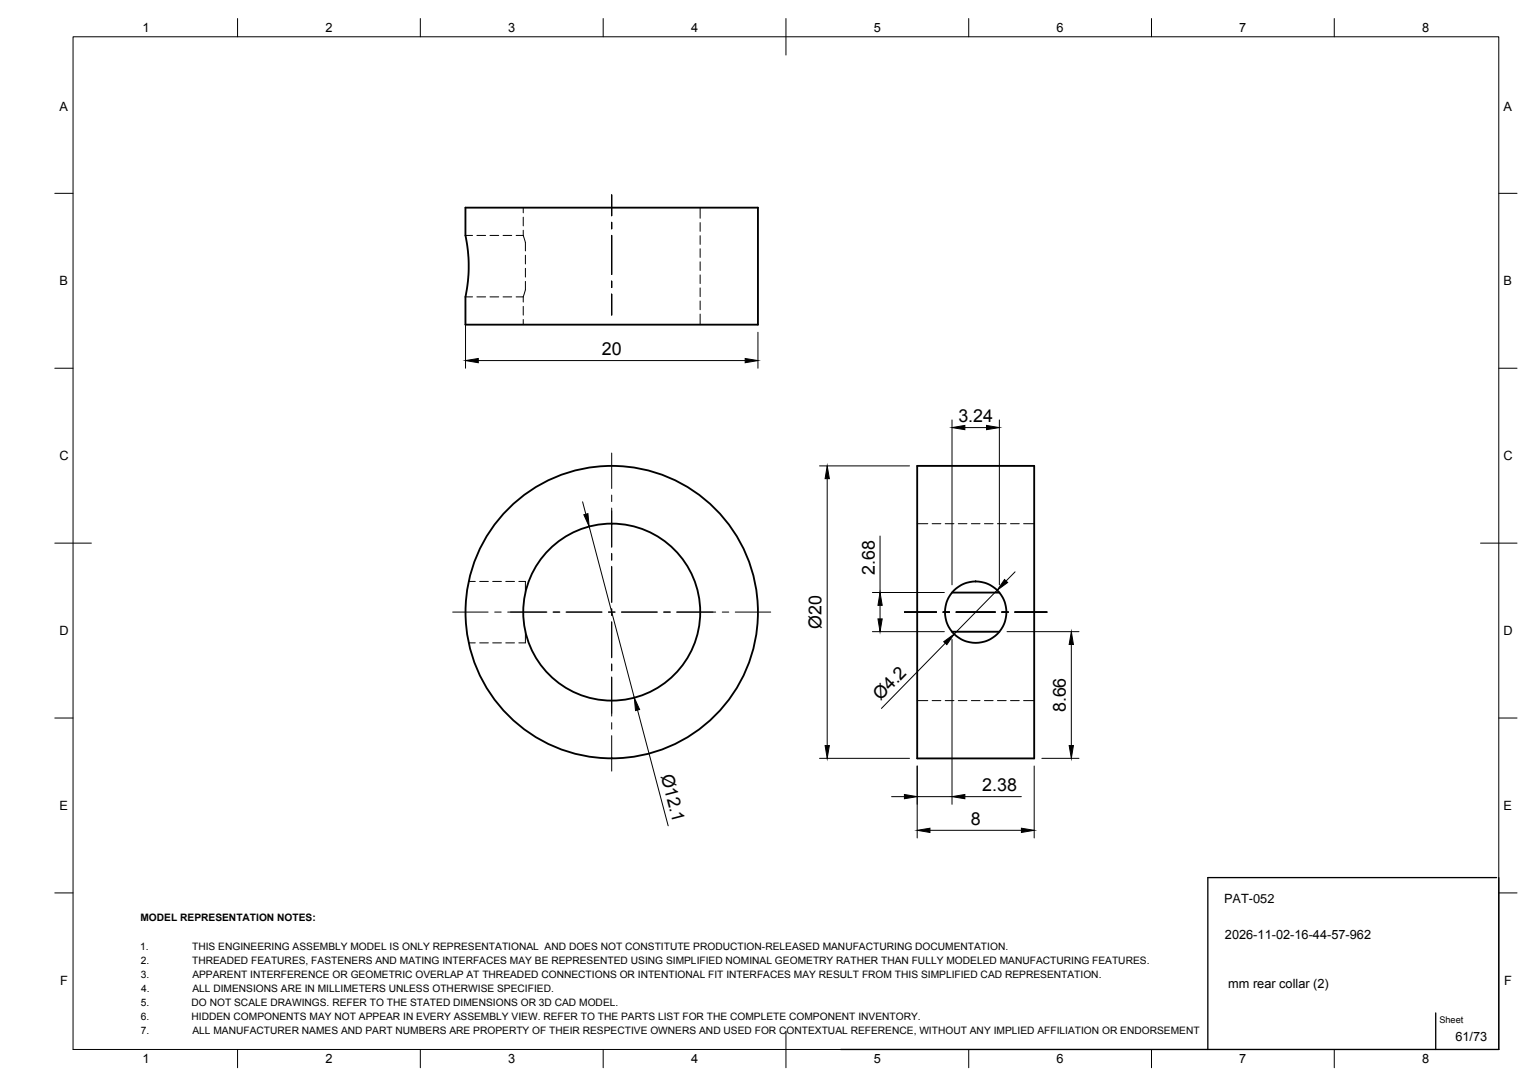
ISO-10303-21;
HEADER;
/* Generated by software containing ST-Developer
 * from STEP Tools, Inc. (www.steptools.com) 
 */

FILE_DESCRIPTION(
/* description */ ('Hand-crank gear train demonstrator'),
/* implementation_level */ '2;1');

FILE_NAME(
/* name */ 'mm rear collar (2).step',
/* time_stamp */ '2026-10-28T03:22:13-07:00',
/* author */ (''),
/* organization */ (''),
/* preprocessor_version */ 'ST-DEVELOPER v20.2',
/* originating_system */ 'Autodesk Translation Framework v15.17.0.0',
/* authorisation */ '');

FILE_SCHEMA (('AUTOMOTIVE_DESIGN { 1 0 10303 214 3 1 1 }'));
ENDSEC;

DATA;
#10=MECHANICAL_DESIGN_GEOMETRIC_PRESENTATION_REPRESENTATION('',(#1251),#62758);
#899=B_SPLINE_CURVE_WITH_KNOTS('',3,(#26683,#26684,#26685,#26686,#26687,
#26688,#26689,#26690,#26691,#26692),.UNSPECIFIED.,.F.,.F.,(4,2,2,2,4),(0.81808890434921,
0.878131747417167,0.957937926194039,1.03774410497091,1.09778694803887),
 .UNSPECIFIED.);
#900=B_SPLINE_CURVE_WITH_KNOTS('',3,(#26698,#26699,#26700,#26701,#26702,
#26703,#26704,#26705,#26706,#26707,#26708,#26709,#26710,#26711,#26712,#26713,
#26714,#26715),.UNSPECIFIED.,.F.,.F.,(4,2,2,2,2,2,2,2,4),(0.,0.0793616477694788,
0.158723295538958,0.238079516586307,0.317435737633657,0.396791958681007,
0.476148179728357,0.555509827497836,0.634871475267315),.UNSPECIFIED.);
#901=B_SPLINE_CURVE_WITH_KNOTS('',3,(#26716,#26717,#26718,#26719,#26720,
#26721,#26722,#26723,#26724,#26725,#26726,#26727,#26728,#26729,#26730,#26731,
#26732,#26733),.UNSPECIFIED.,.F.,.F.,(4,2,2,2,2,2,2,2,4),(0.634871475267315,
0.714233123036793,0.793594770806272,0.872950991853622,0.952307212900972,
1.03166343394832,1.11101965499567,1.19038130276515,1.26974295053463),
 .UNSPECIFIED.);
#902=B_SPLINE_CURVE_WITH_KNOTS('',3,(#26736,#26737,#26738,#26739,#26740,
#26741,#26742,#26743,#26744,#26745),.UNSPECIFIED.,.F.,.F.,(4,2,2,2,4),(0.17946362021985,
0.239506463287808,0.31931264206468,0.399118820841551,0.459161663909509),
 .UNSPECIFIED.);
#1108=SHAPE_REPRESENTATION_RELATIONSHIP('SRR','None',#63085,#1172);
#1172=ADVANCED_BREP_SHAPE_REPRESENTATION('',(#1326),#62739);
#1251=STYLED_ITEM('',(#63448),#1326);
#1326=MANIFOLD_SOLID_BREP('Body1',#16435);
#1594=FACE_BOUND('',#3879,.T.);
#1595=FACE_BOUND('',#3881,.T.);
#1596=FACE_BOUND('',#3883,.T.);
#1597=FACE_BOUND('',#3885,.T.);
#1971=PLANE('',#18248);
#1972=PLANE('',#18253);
#1973=PLANE('',#18260);
#1974=PLANE('',#18261);
#2687=FACE_OUTER_BOUND('',#3875,.T.);
#2688=FACE_OUTER_BOUND('',#3876,.T.);
#2689=FACE_OUTER_BOUND('',#3877,.T.);
#2690=FACE_OUTER_BOUND('',#3878,.T.);
#2691=FACE_OUTER_BOUND('',#3880,.T.);
#2692=FACE_OUTER_BOUND('',#3882,.T.);
#2693=FACE_OUTER_BOUND('',#3884,.T.);
#3875=EDGE_LOOP('',(#13211,#13212));
#3876=EDGE_LOOP('',(#13213,#13214,#13215,#13216,#13217,#13218,#13219,#13220,
#13221));
#3877=EDGE_LOOP('',(#13222,#13223,#13224));
#3878=EDGE_LOOP('',(#13225,#13226,#13227,#13228));
#3879=EDGE_LOOP('',(#13229,#13230,#13231,#13232));
#3880=EDGE_LOOP('',(#13233,#13234,#13235,#13236));
#3881=EDGE_LOOP('',(#13237,#13238));
#3882=EDGE_LOOP('',(#13239));
#3883=EDGE_LOOP('',(#13240));
#3884=EDGE_LOOP('',(#13241));
#3885=EDGE_LOOP('',(#13242));
#4973=LINE('',#26679,#6105);
#4974=LINE('',#26696,#6106);
#4975=LINE('',#26747,#6107);
#4976=LINE('',#26752,#6108);
#4977=LINE('',#26758,#6109);
#6105=VECTOR('',#21700,1.);
#6106=VECTOR('',#21707,0.210000000000001);
#6107=VECTOR('',#21712,1.);
#6108=VECTOR('',#21717,0.605);
#6109=VECTOR('',#21724,1.);
#7011=CIRCLE('',#18249,0.210000000000001);
#7012=CIRCLE('',#18251,0.210000000000001);
#7013=CIRCLE('',#18252,0.210000000000001);
#7014=CIRCLE('',#18255,0.605);
#7015=CIRCLE('',#18256,0.605);
#7016=CIRCLE('',#18258,1.);
#7017=CIRCLE('',#18259,1.);
#8018=VERTEX_POINT('',#26677);
#8019=VERTEX_POINT('',#26678);
#8020=VERTEX_POINT('',#26682);
#8021=VERTEX_POINT('',#26693);
#8022=VERTEX_POINT('',#26695);
#8023=VERTEX_POINT('',#26697);
#8024=VERTEX_POINT('',#26734);
#8025=VERTEX_POINT('',#26749);
#8026=VERTEX_POINT('',#26751);
#8027=VERTEX_POINT('',#26755);
#8028=VERTEX_POINT('',#26757);
#9857=EDGE_CURVE('',#8018,#8019,#4973,.T.);
#9858=EDGE_CURVE('',#8018,#8019,#7011,.T.);
#9859=EDGE_CURVE('',#8020,#8018,#899,.T.);
#9860=EDGE_CURVE('',#8021,#8020,#7012,.T.);
#9861=EDGE_CURVE('',#8021,#8022,#4974,.T.);
#9862=EDGE_CURVE('',#8023,#8022,#900,.T.);
#9863=EDGE_CURVE('',#8022,#8023,#901,.T.);
#9864=EDGE_CURVE('',#8024,#8021,#7013,.T.);
#9865=EDGE_CURVE('',#8019,#8024,#902,.T.);
#9866=EDGE_CURVE('',#8024,#8020,#4975,.T.);
#9867=EDGE_CURVE('',#8025,#8025,#7014,.T.);
#9868=EDGE_CURVE('',#8025,#8026,#4976,.T.);
#9869=EDGE_CURVE('',#8026,#8026,#7015,.T.);
#9870=EDGE_CURVE('',#8027,#8027,#7016,.T.);
#9871=EDGE_CURVE('',#8027,#8028,#4977,.T.);
#9872=EDGE_CURVE('',#8028,#8028,#7017,.T.);
#13211=ORIENTED_EDGE('',*,*,#9857,.F.);
#13212=ORIENTED_EDGE('',*,*,#9858,.T.);
#13213=ORIENTED_EDGE('',*,*,#9859,.F.);
#13214=ORIENTED_EDGE('',*,*,#9860,.F.);
#13215=ORIENTED_EDGE('',*,*,#9861,.T.);
#13216=ORIENTED_EDGE('',*,*,#9862,.F.);
#13217=ORIENTED_EDGE('',*,*,#9863,.F.);
#13218=ORIENTED_EDGE('',*,*,#9861,.F.);
#13219=ORIENTED_EDGE('',*,*,#9864,.F.);
#13220=ORIENTED_EDGE('',*,*,#9865,.F.);
#13221=ORIENTED_EDGE('',*,*,#9858,.F.);
#13222=ORIENTED_EDGE('',*,*,#9866,.F.);
#13223=ORIENTED_EDGE('',*,*,#9864,.T.);
#13224=ORIENTED_EDGE('',*,*,#9860,.T.);
#13225=ORIENTED_EDGE('',*,*,#9867,.F.);
#13226=ORIENTED_EDGE('',*,*,#9868,.T.);
#13227=ORIENTED_EDGE('',*,*,#9869,.T.);
#13228=ORIENTED_EDGE('',*,*,#9868,.F.);
#13229=ORIENTED_EDGE('',*,*,#9865,.T.);
#13230=ORIENTED_EDGE('',*,*,#9866,.T.);
#13231=ORIENTED_EDGE('',*,*,#9859,.T.);
#13232=ORIENTED_EDGE('',*,*,#9857,.T.);
#13233=ORIENTED_EDGE('',*,*,#9870,.F.);
#13234=ORIENTED_EDGE('',*,*,#9871,.T.);
#13235=ORIENTED_EDGE('',*,*,#9872,.T.);
#13236=ORIENTED_EDGE('',*,*,#9871,.F.);
#13237=ORIENTED_EDGE('',*,*,#9862,.T.);
#13238=ORIENTED_EDGE('',*,*,#9863,.T.);
#13239=ORIENTED_EDGE('',*,*,#9870,.T.);
#13240=ORIENTED_EDGE('',*,*,#9867,.T.);
#13241=ORIENTED_EDGE('',*,*,#9872,.F.);
#13242=ORIENTED_EDGE('',*,*,#9869,.F.);
#15339=CYLINDRICAL_SURFACE('',#18250,0.210000000000001);
#15340=CYLINDRICAL_SURFACE('',#18254,0.605);
#15341=CYLINDRICAL_SURFACE('',#18257,1.);
#15997=ADVANCED_FACE('',(#2687),#1971,.T.);
#15998=ADVANCED_FACE('',(#2688),#15339,.F.);
#15999=ADVANCED_FACE('',(#2689),#1972,.T.);
#16000=ADVANCED_FACE('',(#2690,#1594),#15340,.F.);
#16001=ADVANCED_FACE('',(#2691,#1595),#15341,.T.);
#16002=ADVANCED_FACE('',(#2692,#1596),#1973,.T.);
#16003=ADVANCED_FACE('',(#2693,#1597),#1974,.F.);
#16435=CLOSED_SHELL('',(#15997,#15998,#15999,#16000,#16001,#16002,#16003));
#18247=AXIS2_PLACEMENT_3D('',#26675,#21696,#21697);
#18248=AXIS2_PLACEMENT_3D('',#26676,#21698,#21699);
#18249=AXIS2_PLACEMENT_3D('',#26680,#21701,#21702);
#18250=AXIS2_PLACEMENT_3D('',#26681,#21703,#21704);
#18251=AXIS2_PLACEMENT_3D('',#26694,#21705,#21706);
#18252=AXIS2_PLACEMENT_3D('',#26735,#21708,#21709);
#18253=AXIS2_PLACEMENT_3D('',#26746,#21710,#21711);
#18254=AXIS2_PLACEMENT_3D('',#26748,#21713,#21714);
#18255=AXIS2_PLACEMENT_3D('',#26750,#21715,#21716);
#18256=AXIS2_PLACEMENT_3D('',#26753,#21718,#21719);
#18257=AXIS2_PLACEMENT_3D('',#26754,#21720,#21721);
#18258=AXIS2_PLACEMENT_3D('',#26756,#21722,#21723);
#18259=AXIS2_PLACEMENT_3D('',#26759,#21725,#21726);
#18260=AXIS2_PLACEMENT_3D('',#26760,#21727,#21728);
#18261=AXIS2_PLACEMENT_3D('',#26761,#21729,#21730);
#21696=DIRECTION('axis',(0.,0.,1.));
#21697=DIRECTION('refdir',(1.,0.,0.));
#21698=DIRECTION('center_axis',(0.,0.,1.));
#21699=DIRECTION('ref_axis',(1.,0.,0.));
#21700=DIRECTION('',(0.,1.,0.));
#21701=DIRECTION('center_axis',(0.,0.,1.));
#21702=DIRECTION('ref_axis',(1.,0.,0.));
#21703=DIRECTION('center_axis',(0.,0.,1.));
#21704=DIRECTION('ref_axis',(1.,0.,0.));
#21705=DIRECTION('center_axis',(0.,0.,1.));
#21706=DIRECTION('ref_axis',(1.,0.,0.));
#21707=DIRECTION('',(0.,0.,1.));
#21708=DIRECTION('center_axis',(0.,0.,1.));
#21709=DIRECTION('ref_axis',(1.,0.,0.));
#21710=DIRECTION('center_axis',(0.,0.,1.));
#21711=DIRECTION('ref_axis',(1.,0.,0.));
#21712=DIRECTION('',(0.,-1.,0.));
#21713=DIRECTION('center_axis',(0.,1.,0.));
#21714=DIRECTION('ref_axis',(1.,0.,0.));
#21715=DIRECTION('center_axis',(0.,-1.,0.));
#21716=DIRECTION('ref_axis',(1.,0.,0.));
#21717=DIRECTION('',(0.,-1.,0.));
#21718=DIRECTION('center_axis',(0.,-1.,0.));
#21719=DIRECTION('ref_axis',(1.,0.,0.));
#21720=DIRECTION('center_axis',(0.,1.,0.));
#21721=DIRECTION('ref_axis',(1.,0.,0.));
#21722=DIRECTION('center_axis',(0.,1.,0.));
#21723=DIRECTION('ref_axis',(1.,0.,0.));
#21724=DIRECTION('',(0.,-1.,0.));
#21725=DIRECTION('center_axis',(0.,1.,0.));
#21726=DIRECTION('ref_axis',(1.,0.,0.));
#21727=DIRECTION('center_axis',(0.,1.,0.));
#21728=DIRECTION('ref_axis',(1.,0.,0.));
#21729=DIRECTION('center_axis',(0.,1.,0.));
#21730=DIRECTION('ref_axis',(1.,0.,0.));
#26675=CARTESIAN_POINT('',(0.,0.,0.));
#26676=CARTESIAN_POINT('Origin',(12.,-3.2,9.59));
#26677=CARTESIAN_POINT('',(12.1338842783899,-3.36178689687366,9.59));
#26678=CARTESIAN_POINT('',(12.1338842783899,-3.03821310312634,9.59));
#26679=CARTESIAN_POINT('',(12.13388427839,-3.6,9.59));
#26680=CARTESIAN_POINT('Origin',(12.,-3.2,9.59));
#26681=CARTESIAN_POINT('Origin',(12.,-3.2,9.59));
#26682=CARTESIAN_POINT('',(11.8661157216101,-3.36178689687366,9.59));
#26683=CARTESIAN_POINT('Ctrl Pts',(11.8661157216101,-3.36178689687366,9.59000000000001));
#26684=CARTESIAN_POINT('Ctrl Pts',(11.8817456047392,-3.37472116821764,9.59354677224418));
#26685=CARTESIAN_POINT('Ctrl Pts',(11.8998902123177,-3.38579931658744,9.59698224789958));
#26686=CARTESIAN_POINT('Ctrl Pts',(11.9451701278675,-3.40463856105443,9.60307416289971));
#26687=CARTESIAN_POINT('Ctrl Pts',(11.9733979404077,-3.41,9.605));
#26688=CARTESIAN_POINT('Ctrl Pts',(12.0266020595923,-3.41,9.605));
#26689=CARTESIAN_POINT('Ctrl Pts',(12.0548298721325,-3.40463856105443,9.60307416289971));
#26690=CARTESIAN_POINT('Ctrl Pts',(12.1001097876823,-3.38579931658744,9.59698224789958));
#26691=CARTESIAN_POINT('Ctrl Pts',(12.1182543952608,-3.37472116821764,9.59354677224418));
#26692=CARTESIAN_POINT('Ctrl Pts',(12.1338842783899,-3.36178689687366,9.59000000000001));
#26693=CARTESIAN_POINT('',(11.79,-3.2,9.59));
#26694=CARTESIAN_POINT('Origin',(12.,-3.2,9.59));
#26695=CARTESIAN_POINT('',(11.79,-3.2,9.97770138590471));
#26696=CARTESIAN_POINT('',(11.79,-3.2,9.59));
#26697=CARTESIAN_POINT('',(12.21,-3.2,9.97770138590471));
#26698=CARTESIAN_POINT('Ctrl Pts',(12.21,-3.2,9.97770138590471));
#26699=CARTESIAN_POINT('Ctrl Pts',(12.21,-3.22645388258983,9.97770138590471));
#26700=CARTESIAN_POINT('Ctrl Pts',(12.2046970171255,-3.25461525830869,9.97888646613217));
#26701=CARTESIAN_POINT('Ctrl Pts',(12.1832417515155,-3.30633042130174,9.98312869991148));
#26702=CARTESIAN_POINT('Ctrl Pts',(12.1670935868029,-3.32989126129544,9.98612044796649));
#26703=CARTESIAN_POINT('Ctrl Pts',(12.1298925332365,-3.36709231486181,9.99170645156379));
#26704=CARTESIAN_POINT('Ctrl Pts',(12.1063311549927,-3.38324147510569,9.99466914446598));
#26705=CARTESIAN_POINT('Ctrl Pts',(12.0546141143984,-3.40469746372443,9.99884449237241));
#26706=CARTESIAN_POINT('Ctrl Pts',(12.0264520736824,-3.41,10.));
#26707=CARTESIAN_POINT('Ctrl Pts',(11.9735479263176,-3.41,10.));
#26708=CARTESIAN_POINT('Ctrl Pts',(11.9453858856017,-3.40469746372443,9.99884449237241));
#26709=CARTESIAN_POINT('Ctrl Pts',(11.8936688450073,-3.38324147510569,9.99466914446598));
#26710=CARTESIAN_POINT('Ctrl Pts',(11.8701074667635,-3.36709231486181,9.99170645156379));
#26711=CARTESIAN_POINT('Ctrl Pts',(11.8329064131971,-3.32989126129544,9.98612044796649));
#26712=CARTESIAN_POINT('Ctrl Pts',(11.8167582484845,-3.30633042130174,9.98312869991148));
#26713=CARTESIAN_POINT('Ctrl Pts',(11.7953029828745,-3.25461525830869,9.97888646613217));
#26714=CARTESIAN_POINT('Ctrl Pts',(11.79,-3.22645388258983,9.97770138590472));
#26715=CARTESIAN_POINT('Ctrl Pts',(11.79,-3.2,9.97770138590472));
#26716=CARTESIAN_POINT('Ctrl Pts',(11.79,-3.2,9.97770138590471));
#26717=CARTESIAN_POINT('Ctrl Pts',(11.79,-3.17354611741017,9.97770138590471));
#26718=CARTESIAN_POINT('Ctrl Pts',(11.7953029828745,-3.14538474169131,9.97888646613217));
#26719=CARTESIAN_POINT('Ctrl Pts',(11.8167582484845,-3.09366957869826,9.98312869991148));
#26720=CARTESIAN_POINT('Ctrl Pts',(11.8329064131971,-3.07010873870456,9.98612044796649));
#26721=CARTESIAN_POINT('Ctrl Pts',(11.8701074667635,-3.03290768513819,9.99170645156379));
#26722=CARTESIAN_POINT('Ctrl Pts',(11.8936688450073,-3.01675852489431,9.99466914446598));
#26723=CARTESIAN_POINT('Ctrl Pts',(11.9453858856016,-2.99530253627557,9.99884449237241));
#26724=CARTESIAN_POINT('Ctrl Pts',(11.9735479263176,-2.99,10.));
#26725=CARTESIAN_POINT('Ctrl Pts',(12.0264520736824,-2.99,10.));
#26726=CARTESIAN_POINT('Ctrl Pts',(12.0546141143984,-2.99530253627557,9.99884449237241));
#26727=CARTESIAN_POINT('Ctrl Pts',(12.1063311549927,-3.01675852489431,9.99466914446598));
#26728=CARTESIAN_POINT('Ctrl Pts',(12.1298925332365,-3.03290768513819,9.99170645156379));
#26729=CARTESIAN_POINT('Ctrl Pts',(12.1670935868029,-3.07010873870456,9.98612044796649));
#26730=CARTESIAN_POINT('Ctrl Pts',(12.1832417515155,-3.09366957869826,9.98312869991147));
#26731=CARTESIAN_POINT('Ctrl Pts',(12.2046970171255,-3.14538474169131,9.97888646613217));
#26732=CARTESIAN_POINT('Ctrl Pts',(12.21,-3.17354611741017,9.97770138590471));
#26733=CARTESIAN_POINT('Ctrl Pts',(12.21,-3.2,9.97770138590471));
#26734=CARTESIAN_POINT('',(11.8661157216101,-3.03821310312634,9.59));
#26735=CARTESIAN_POINT('Origin',(12.,-3.2,9.59));
#26736=CARTESIAN_POINT('Ctrl Pts',(12.1338842783899,-3.03821310312634,9.59000000000001));
#26737=CARTESIAN_POINT('Ctrl Pts',(12.1182543952608,-3.02527883178236,9.59354677224418));
#26738=CARTESIAN_POINT('Ctrl Pts',(12.1001097876823,-3.01420068341256,9.59698224789958));
#26739=CARTESIAN_POINT('Ctrl Pts',(12.0548298721325,-2.99536143894557,9.60307416289971));
#26740=CARTESIAN_POINT('Ctrl Pts',(12.0266020595923,-2.99,9.605));
#26741=CARTESIAN_POINT('Ctrl Pts',(11.9733979404077,-2.99,9.605));
#26742=CARTESIAN_POINT('Ctrl Pts',(11.9451701278675,-2.99536143894557,9.60307416289971));
#26743=CARTESIAN_POINT('Ctrl Pts',(11.8998902123177,-3.01420068341256,9.59698224789958));
#26744=CARTESIAN_POINT('Ctrl Pts',(11.8817456047392,-3.02527883178236,9.59354677224418));
#26745=CARTESIAN_POINT('Ctrl Pts',(11.8661157216101,-3.03821310312634,9.59000000000001));
#26746=CARTESIAN_POINT('Origin',(12.,-3.2,9.59));
#26747=CARTESIAN_POINT('',(11.86611572161,-3.6,9.59));
#26748=CARTESIAN_POINT('Origin',(12.,-3.6,9.));
#26749=CARTESIAN_POINT('',(11.395,-2.8,9.));
#26750=CARTESIAN_POINT('Origin',(12.,-2.8,9.));
#26751=CARTESIAN_POINT('',(11.395,-3.6,9.));
#26752=CARTESIAN_POINT('',(11.395,-3.6,9.));
#26753=CARTESIAN_POINT('Origin',(12.,-3.6,9.));
#26754=CARTESIAN_POINT('Origin',(12.,-3.6,9.));
#26755=CARTESIAN_POINT('',(11.,-2.8,9.));
#26756=CARTESIAN_POINT('Origin',(12.,-2.8,9.));
#26757=CARTESIAN_POINT('',(11.,-3.6,9.));
#26758=CARTESIAN_POINT('',(11.,-3.6,9.));
#26759=CARTESIAN_POINT('Origin',(12.,-3.6,9.));
#26760=CARTESIAN_POINT('Origin',(12.,-2.8,9.));
#26761=CARTESIAN_POINT('Origin',(12.,-3.6,9.));
#62665=UNCERTAINTY_MEASURE_WITH_UNIT(LENGTH_MEASURE(0.001),#62759,
'DISTANCE_ACCURACY_VALUE',
'Maximum model space distance between geometric entities at asserted c
onnectivities');
#62684=UNCERTAINTY_MEASURE_WITH_UNIT(LENGTH_MEASURE(0.001),#62759,
'DISTANCE_ACCURACY_VALUE',
'Maximum model space distance between geometric entities at asserted c
onnectivities');
#62739=(
GEOMETRIC_REPRESENTATION_CONTEXT(3)
GLOBAL_UNCERTAINTY_ASSIGNED_CONTEXT((#62665))
GLOBAL_UNIT_ASSIGNED_CONTEXT((#62759,#62761,#62762))
REPRESENTATION_CONTEXT('','3D')
);
#62758=(
GEOMETRIC_REPRESENTATION_CONTEXT(3)
GLOBAL_UNCERTAINTY_ASSIGNED_CONTEXT((#62684))
GLOBAL_UNIT_ASSIGNED_CONTEXT((#62759,#62761,#62762))
REPRESENTATION_CONTEXT('','3D')
);
#62759=(
LENGTH_UNIT()
NAMED_UNIT(*)
SI_UNIT(.CENTI.,.METRE.)
);
#62761=(
NAMED_UNIT(*)
PLANE_ANGLE_UNIT()
SI_UNIT($,.RADIAN.)
);
#62762=(
NAMED_UNIT(*)
SI_UNIT($,.STERADIAN.)
SOLID_ANGLE_UNIT()
);
#62817=SHAPE_DEFINITION_REPRESENTATION(#62900,#63085);
#62900=PRODUCT_DEFINITION_SHAPE('',$,#63159);
#63085=SHAPE_REPRESENTATION('',(#18247),#62739);
#63104=PRODUCT_DEFINITION_CONTEXT('part definition',#63325,'design');
#63159=PRODUCT_DEFINITION('mm rear collar (2)','mm rear collar (2)',#63232,
#63104);
#63232=PRODUCT_DEFINITION_FORMATION('',$,#63381);
#63325=APPLICATION_CONTEXT(
'Core Data for Automotive Mechanical Design Process');
#63326=PRODUCT_CONTEXT('part definition',#63325,'mechanical');
#63381=PRODUCT('mm rear collar (2)','mm rear collar (2)','mm rear collar (2)',
(#63326));
#63442=COLOUR_RGB('Light Blue',0.38,0.62,0.78);
#63443=FILL_AREA_STYLE_COLOUR('',#63442);
#63444=FILL_AREA_STYLE('',(#63443));
#63445=SURFACE_STYLE_FILL_AREA(#63444);
#63446=SURFACE_SIDE_STYLE('',(#63445));
#63447=SURFACE_STYLE_USAGE(.BOTH.,#63446);
#63448=PRESENTATION_STYLE_ASSIGNMENT((#63447));
ENDSEC;
END-ISO-10303-21;
